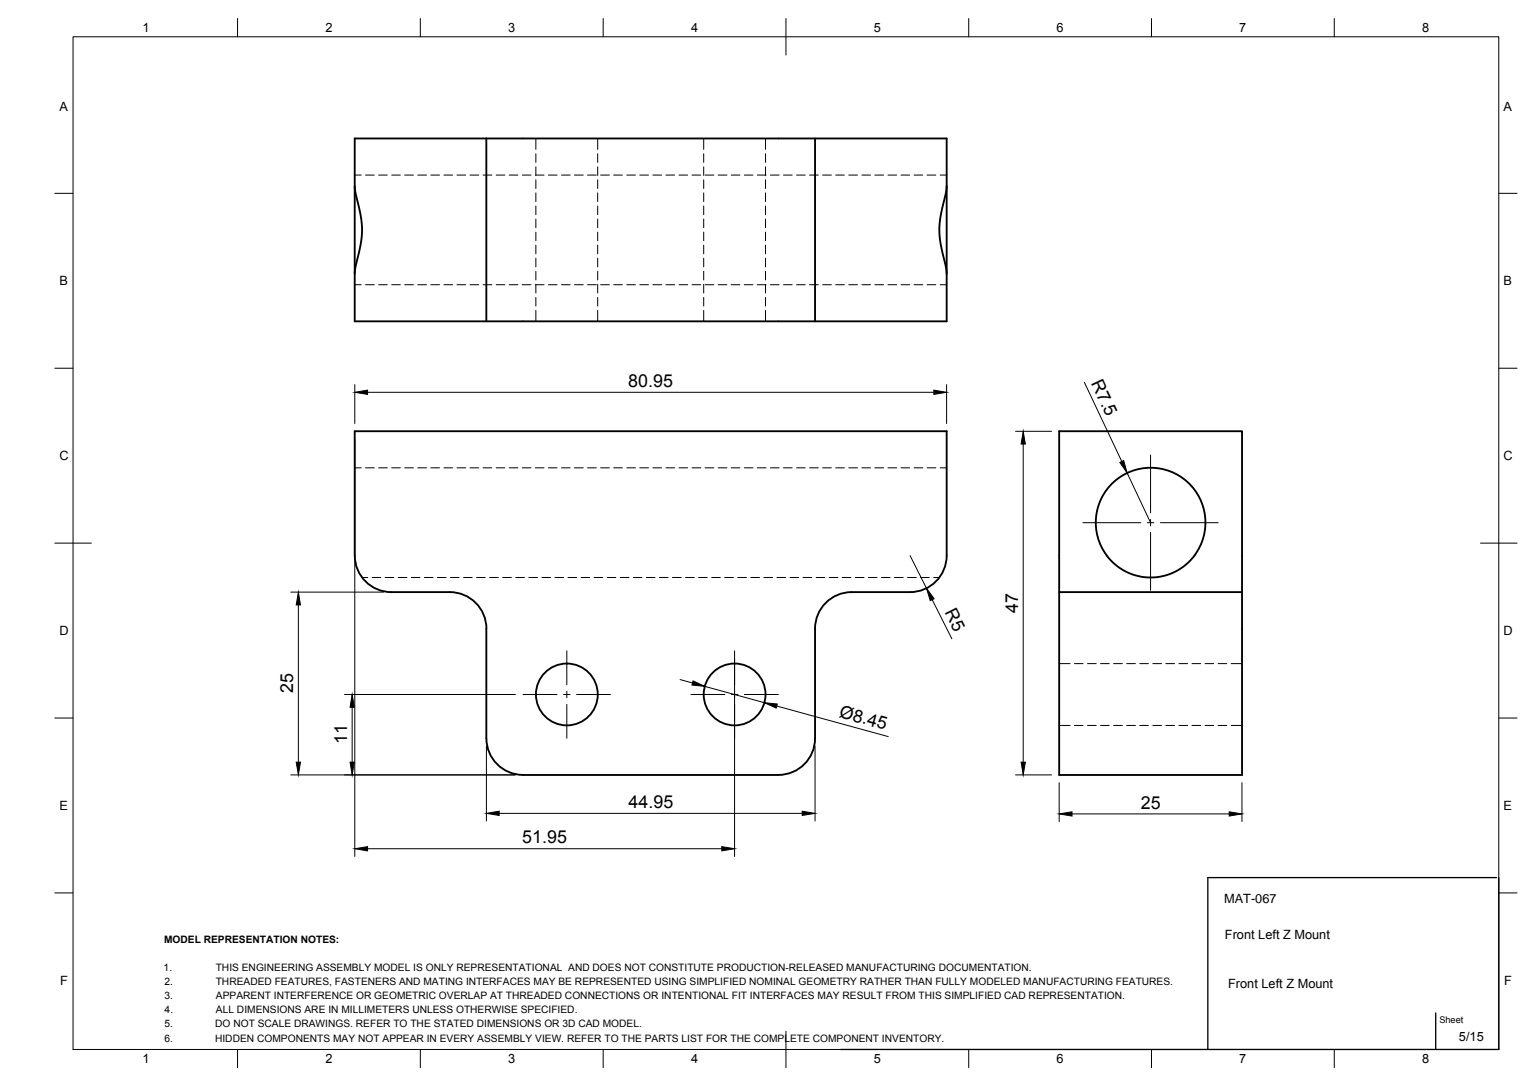
ISO-10303-21;
HEADER;
/* Generated by software containing ST-Developer
 * from STEP Tools, Inc. (www.steptools.com) 
 */

FILE_DESCRIPTION(
/* description */ ('CAx-IF Rec.Pracs.---Representation and Presentation of Product Manufa
cturing Information (PMI)---4.0---2014-10-13'),
/* implementation_level */ '2;1');

FILE_NAME(
/* name */ 'Front Left Z Mount.step',
/* time_stamp */ '2026-10-24T16:02:03-07:00',
/* author */ (''),
/* organization */ (''),
/* preprocessor_version */ 'ST-DEVELOPER v20.2',
/* originating_system */ 'Autodesk Translation Framework v15.17.0.0',
/* authorisation */ '');

FILE_SCHEMA (('AP242_MANAGED_MODEL_BASED_3D_ENGINEERING_MIM_LF { 1 0 10303 442 2 1 4 }'));
ENDSEC;

DATA;
#10=MECHANICAL_DESIGN_GEOMETRIC_PRESENTATION_REPRESENTATION('',(#351),#6348);
#329=SHAPE_REPRESENTATION_RELATIONSHIP('SRR','None',#6479,#340);
#340=ADVANCED_BREP_SHAPE_REPRESENTATION('',(#362),#6327);
#351=STYLED_ITEM('',(#6602),#362);
#362=MANIFOLD_SOLID_BREP('Body1',#3390);
#375=B_SPLINE_CURVE_WITH_KNOTS('',3,(#5524,#5525,#5526,#5527,#5528,#5529,
#5530,#5531,#5532,#5533,#5534,#5535,#5536,#5537,#5538,#5539,#5540,#5541),
 .UNSPECIFIED.,.F.,.F.,(4,2,2,2,2,2,2,2,4),(-2.14352388719531,-2.06484634554612,
-1.76300355616504,-1.61208216147449,-1.46116076678395,-1.31023937209341,
-1.15931797740286,-0.857475188021775,-0.778797646372586),.UNSPECIFIED.);
#376=B_SPLINE_CURVE_WITH_KNOTS('',3,(#5543,#5544,#5545,#5546,#5547,#5548,
#5549,#5550,#5551,#5552,#5553,#5554,#5555,#5556,#5557,#5558,#5559,#5560),
 .UNSPECIFIED.,.F.,.F.,(4,2,2,2,2,2,2,2,4),(-5.06584542076321,-4.98716787911402,
-4.68532508973293,-4.53440369504239,-4.38348230035184,-4.2325609056613,
-4.08163951097076,-3.77979672158967,-3.70111917994048),.UNSPECIFIED.);
#403=CYLINDRICAL_SURFACE('',#3628,0.004225);
#404=CYLINDRICAL_SURFACE('',#3629,0.004225);
#405=CYLINDRICAL_SURFACE('',#3631,0.0075);
#406=CYLINDRICAL_SURFACE('',#3636,0.005);
#407=CYLINDRICAL_SURFACE('',#3637,0.005);
#408=CYLINDRICAL_SURFACE('',#3638,0.005);
#409=CYLINDRICAL_SURFACE('',#3639,0.005);
#410=CYLINDRICAL_SURFACE('',#3640,0.005);
#411=CYLINDRICAL_SURFACE('',#3641,0.005);
#472=FACE_BOUND('',#915,.T.);
#473=FACE_BOUND('',#916,.T.);
#474=FACE_BOUND('',#918,.T.);
#475=FACE_BOUND('',#919,.T.);
#546=CIRCLE('',#3605,0.0075);
#547=CIRCLE('',#3606,0.0075);
#548=CIRCLE('',#3608,0.0075);
#549=CIRCLE('',#3609,0.0075);
#550=CIRCLE('',#3611,0.005);
#551=CIRCLE('',#3612,0.005);
#552=CIRCLE('',#3613,0.005);
#553=CIRCLE('',#3614,0.005);
#554=CIRCLE('',#3615,0.005);
#555=CIRCLE('',#3616,0.005);
#556=CIRCLE('',#3617,0.004225);
#557=CIRCLE('',#3618,0.004225);
#558=CIRCLE('',#3620,0.005);
#559=CIRCLE('',#3621,0.005);
#560=CIRCLE('',#3622,0.005);
#561=CIRCLE('',#3623,0.005);
#562=CIRCLE('',#3624,0.005);
#563=CIRCLE('',#3625,0.005);
#564=CIRCLE('',#3626,0.004225);
#565=CIRCLE('',#3627,0.004225);
#732=FACE_OUTER_BOUND('',#911,.T.);
#733=FACE_OUTER_BOUND('',#912,.T.);
#734=FACE_OUTER_BOUND('',#913,.T.);
#735=FACE_OUTER_BOUND('',#914,.T.);
#736=FACE_OUTER_BOUND('',#917,.T.);
#737=FACE_OUTER_BOUND('',#920,.T.);
#738=FACE_OUTER_BOUND('',#921,.T.);
#739=FACE_OUTER_BOUND('',#922,.T.);
#740=FACE_OUTER_BOUND('',#923,.T.);
#741=FACE_OUTER_BOUND('',#924,.T.);
#742=FACE_OUTER_BOUND('',#925,.T.);
#743=FACE_OUTER_BOUND('',#926,.T.);
#744=FACE_OUTER_BOUND('',#927,.T.);
#745=FACE_OUTER_BOUND('',#928,.T.);
#746=FACE_OUTER_BOUND('',#929,.T.);
#747=FACE_OUTER_BOUND('',#930,.T.);
#748=FACE_OUTER_BOUND('',#931,.T.);
#749=FACE_OUTER_BOUND('',#932,.T.);
#750=FACE_OUTER_BOUND('',#933,.T.);
#911=EDGE_LOOP('',(#2495,#2496,#2497,#2498));
#912=EDGE_LOOP('',(#2499,#2500,#2501,#2502,#2503,#2504,#2505));
#913=EDGE_LOOP('',(#2506,#2507,#2508,#2509,#2510,#2511,#2512));
#914=EDGE_LOOP('',(#2513,#2514,#2515,#2516,#2517,#2518,#2519,#2520,#2521,
#2522,#2523,#2524,#2525,#2526));
#915=EDGE_LOOP('',(#2527));
#916=EDGE_LOOP('',(#2528));
#917=EDGE_LOOP('',(#2529,#2530,#2531,#2532,#2533,#2534,#2535,#2536,#2537,
#2538,#2539,#2540,#2541,#2542));
#918=EDGE_LOOP('',(#2543));
#919=EDGE_LOOP('',(#2544));
#920=EDGE_LOOP('',(#2545,#2546,#2547,#2548));
#921=EDGE_LOOP('',(#2549,#2550,#2551,#2552));
#922=EDGE_LOOP('',(#2553,#2554,#2555,#2556));
#923=EDGE_LOOP('',(#2557,#2558,#2559,#2560,#2561,#2562,#2563,#2564));
#924=EDGE_LOOP('',(#2565,#2566,#2567,#2568));
#925=EDGE_LOOP('',(#2569,#2570,#2571,#2572));
#926=EDGE_LOOP('',(#2573,#2574,#2575,#2576));
#927=EDGE_LOOP('',(#2577,#2578,#2579,#2580));
#928=EDGE_LOOP('',(#2581,#2582,#2583,#2584));
#929=EDGE_LOOP('',(#2585,#2586,#2587,#2588,#2589,#2590));
#930=EDGE_LOOP('',(#2591,#2592,#2593,#2594));
#931=EDGE_LOOP('',(#2595,#2596,#2597,#2598,#2599,#2600));
#932=EDGE_LOOP('',(#2601,#2602,#2603,#2604));
#933=EDGE_LOOP('',(#2605,#2606,#2607,#2608));
#1148=LINE('',#5434,#1381);
#1149=LINE('',#5436,#1382);
#1150=LINE('',#5438,#1383);
#1151=LINE('',#5439,#1384);
#1152=LINE('',#5443,#1385);
#1153=LINE('',#5445,#1386);
#1154=LINE('',#5451,#1387);
#1155=LINE('',#5453,#1388);
#1156=LINE('',#5454,#1389);
#1157=LINE('',#5458,#1390);
#1158=LINE('',#5460,#1391);
#1159=LINE('',#5466,#1392);
#1160=LINE('',#5468,#1393);
#1161=LINE('',#5469,#1394);
#1162=LINE('',#5474,#1395);
#1163=LINE('',#5478,#1396);
#1164=LINE('',#5480,#1397);
#1165=LINE('',#5484,#1398);
#1166=LINE('',#5488,#1399);
#1167=LINE('',#5497,#1400);
#1168=LINE('',#5502,#1401);
#1169=LINE('',#5506,#1402);
#1170=LINE('',#5508,#1403);
#1171=LINE('',#5512,#1404);
#1172=LINE('',#5519,#1405);
#1173=LINE('',#5521,#1406);
#1174=LINE('',#5542,#1407);
#1175=LINE('',#5562,#1408);
#1176=LINE('',#5563,#1409);
#1177=LINE('',#5565,#1410);
#1178=LINE('',#5566,#1411);
#1179=LINE('',#5568,#1412);
#1180=LINE('',#5569,#1413);
#1181=LINE('',#5571,#1414);
#1182=LINE('',#5572,#1415);
#1381=VECTOR('',#4216,1.);
#1382=VECTOR('',#4217,1.);
#1383=VECTOR('',#4218,1.);
#1384=VECTOR('',#4219,1.);
#1385=VECTOR('',#4222,1.);
#1386=VECTOR('',#4223,1.);
#1387=VECTOR('',#4228,1.);
#1388=VECTOR('',#4229,1.);
#1389=VECTOR('',#4230,1.);
#1390=VECTOR('',#4233,1.);
#1391=VECTOR('',#4234,1.);
#1392=VECTOR('',#4239,1.);
#1393=VECTOR('',#4240,1.);
#1394=VECTOR('',#4241,1.);
#1395=VECTOR('',#4246,1.);
#1396=VECTOR('',#4249,1.);
#1397=VECTOR('',#4252,1.);
#1398=VECTOR('',#4255,1.);
#1399=VECTOR('',#4258,1.);
#1400=VECTOR('',#4267,1.);
#1401=VECTOR('',#4272,1.);
#1402=VECTOR('',#4275,1.);
#1403=VECTOR('',#4278,1.);
#1404=VECTOR('',#4281,1.);
#1405=VECTOR('',#4290,0.004225);
#1406=VECTOR('',#4293,0.004225);
#1407=VECTOR('',#4298,0.0075);
#1408=VECTOR('',#4301,1.);
#1409=VECTOR('',#4302,1.);
#1410=VECTOR('',#4305,1.);
#1411=VECTOR('',#4306,1.);
#1412=VECTOR('',#4309,1.);
#1413=VECTOR('',#4310,1.);
#1414=VECTOR('',#4313,1.);
#1415=VECTOR('',#4314,1.);
#1620=VERTEX_POINT('',#5432);
#1621=VERTEX_POINT('',#5433);
#1622=VERTEX_POINT('',#5435);
#1623=VERTEX_POINT('',#5437);
#1624=VERTEX_POINT('',#5441);
#1625=VERTEX_POINT('',#5442);
#1626=VERTEX_POINT('',#5444);
#1627=VERTEX_POINT('',#5446);
#1628=VERTEX_POINT('',#5448);
#1629=VERTEX_POINT('',#5450);
#1630=VERTEX_POINT('',#5452);
#1631=VERTEX_POINT('',#5456);
#1632=VERTEX_POINT('',#5457);
#1633=VERTEX_POINT('',#5459);
#1634=VERTEX_POINT('',#5461);
#1635=VERTEX_POINT('',#5463);
#1636=VERTEX_POINT('',#5465);
#1637=VERTEX_POINT('',#5467);
#1638=VERTEX_POINT('',#5471);
#1639=VERTEX_POINT('',#5473);
#1640=VERTEX_POINT('',#5475);
#1641=VERTEX_POINT('',#5477);
#1642=VERTEX_POINT('',#5481);
#1643=VERTEX_POINT('',#5483);
#1644=VERTEX_POINT('',#5485);
#1645=VERTEX_POINT('',#5487);
#1646=VERTEX_POINT('',#5490);
#1647=VERTEX_POINT('',#5492);
#1648=VERTEX_POINT('',#5495);
#1649=VERTEX_POINT('',#5496);
#1650=VERTEX_POINT('',#5499);
#1651=VERTEX_POINT('',#5501);
#1652=VERTEX_POINT('',#5503);
#1653=VERTEX_POINT('',#5505);
#1654=VERTEX_POINT('',#5509);
#1655=VERTEX_POINT('',#5511);
#1656=VERTEX_POINT('',#5514);
#1657=VERTEX_POINT('',#5516);
#1946=EDGE_CURVE('',#1620,#1621,#1148,.T.);
#1947=EDGE_CURVE('',#1621,#1622,#1149,.T.);
#1948=EDGE_CURVE('',#1623,#1622,#1150,.T.);
#1949=EDGE_CURVE('',#1623,#1620,#1151,.F.);
#1950=EDGE_CURVE('',#1624,#1625,#1152,.T.);
#1951=EDGE_CURVE('',#1624,#1626,#1153,.F.);
#1952=EDGE_CURVE('',#1626,#1627,#546,.T.);
#1953=EDGE_CURVE('',#1627,#1628,#547,.T.);
#1954=EDGE_CURVE('',#1628,#1629,#1154,.F.);
#1955=EDGE_CURVE('',#1629,#1630,#1155,.T.);
#1956=EDGE_CURVE('',#1625,#1630,#1156,.T.);
#1957=EDGE_CURVE('',#1631,#1632,#1157,.T.);
#1958=EDGE_CURVE('',#1631,#1633,#1158,.T.);
#1959=EDGE_CURVE('',#1634,#1633,#548,.T.);
#1960=EDGE_CURVE('',#1635,#1634,#549,.T.);
#1961=EDGE_CURVE('',#1635,#1636,#1159,.T.);
#1962=EDGE_CURVE('',#1636,#1637,#1160,.T.);
#1963=EDGE_CURVE('',#1637,#1632,#1161,.T.);
#1964=EDGE_CURVE('',#1622,#1638,#550,.T.);
#1965=EDGE_CURVE('',#1638,#1639,#1162,.T.);
#1966=EDGE_CURVE('',#1639,#1640,#551,.F.);
#1967=EDGE_CURVE('',#1641,#1640,#1163,.T.);
#1968=EDGE_CURVE('',#1641,#1624,#552,.T.);
#1969=EDGE_CURVE('',#1637,#1625,#1164,.T.);
#1970=EDGE_CURVE('',#1636,#1642,#553,.T.);
#1971=EDGE_CURVE('',#1642,#1643,#1165,.T.);
#1972=EDGE_CURVE('',#1643,#1644,#554,.F.);
#1973=EDGE_CURVE('',#1645,#1644,#1166,.T.);
#1974=EDGE_CURVE('',#1645,#1623,#555,.T.);
#1975=EDGE_CURVE('',#1646,#1646,#556,.T.);
#1976=EDGE_CURVE('',#1647,#1647,#557,.T.);
#1977=EDGE_CURVE('',#1648,#1649,#1167,.T.);
#1978=EDGE_CURVE('',#1648,#1621,#558,.F.);
#1979=EDGE_CURVE('',#1620,#1650,#559,.F.);
#1980=EDGE_CURVE('',#1650,#1651,#1168,.T.);
#1981=EDGE_CURVE('',#1651,#1652,#560,.T.);
#1982=EDGE_CURVE('',#1653,#1652,#1169,.T.);
#1983=EDGE_CURVE('',#1653,#1631,#561,.F.);
#1984=EDGE_CURVE('',#1632,#1630,#1170,.T.);
#1985=EDGE_CURVE('',#1629,#1654,#562,.F.);
#1986=EDGE_CURVE('',#1654,#1655,#1171,.T.);
#1987=EDGE_CURVE('',#1655,#1649,#563,.T.);
#1988=EDGE_CURVE('',#1656,#1656,#564,.T.);
#1989=EDGE_CURVE('',#1657,#1657,#565,.T.);
#1990=EDGE_CURVE('',#1646,#1656,#1172,.T.);
#1991=EDGE_CURVE('',#1647,#1657,#1173,.T.);
#1992=EDGE_CURVE('',#1626,#1628,#375,.T.);
#1993=EDGE_CURVE('',#1627,#1634,#1174,.T.);
#1994=EDGE_CURVE('',#1633,#1635,#376,.T.);
#1995=EDGE_CURVE('',#1638,#1648,#1175,.F.);
#1996=EDGE_CURVE('',#1649,#1639,#1176,.T.);
#1997=EDGE_CURVE('',#1654,#1641,#1177,.T.);
#1998=EDGE_CURVE('',#1640,#1655,#1178,.F.);
#1999=EDGE_CURVE('',#1644,#1651,#1179,.F.);
#2000=EDGE_CURVE('',#1650,#1645,#1180,.T.);
#2001=EDGE_CURVE('',#1642,#1653,#1181,.F.);
#2002=EDGE_CURVE('',#1652,#1643,#1182,.T.);
#2495=ORIENTED_EDGE('',*,*,#1946,.T.);
#2496=ORIENTED_EDGE('',*,*,#1947,.T.);
#2497=ORIENTED_EDGE('',*,*,#1948,.F.);
#2498=ORIENTED_EDGE('',*,*,#1949,.T.);
#2499=ORIENTED_EDGE('',*,*,#1950,.F.);
#2500=ORIENTED_EDGE('',*,*,#1951,.T.);
#2501=ORIENTED_EDGE('',*,*,#1952,.T.);
#2502=ORIENTED_EDGE('',*,*,#1953,.T.);
#2503=ORIENTED_EDGE('',*,*,#1954,.T.);
#2504=ORIENTED_EDGE('',*,*,#1955,.T.);
#2505=ORIENTED_EDGE('',*,*,#1956,.F.);
#2506=ORIENTED_EDGE('',*,*,#1957,.F.);
#2507=ORIENTED_EDGE('',*,*,#1958,.T.);
#2508=ORIENTED_EDGE('',*,*,#1959,.F.);
#2509=ORIENTED_EDGE('',*,*,#1960,.F.);
#2510=ORIENTED_EDGE('',*,*,#1961,.T.);
#2511=ORIENTED_EDGE('',*,*,#1962,.T.);
#2512=ORIENTED_EDGE('',*,*,#1963,.T.);
#2513=ORIENTED_EDGE('',*,*,#1948,.T.);
#2514=ORIENTED_EDGE('',*,*,#1964,.T.);
#2515=ORIENTED_EDGE('',*,*,#1965,.T.);
#2516=ORIENTED_EDGE('',*,*,#1966,.T.);
#2517=ORIENTED_EDGE('',*,*,#1967,.F.);
#2518=ORIENTED_EDGE('',*,*,#1968,.T.);
#2519=ORIENTED_EDGE('',*,*,#1950,.T.);
#2520=ORIENTED_EDGE('',*,*,#1969,.F.);
#2521=ORIENTED_EDGE('',*,*,#1962,.F.);
#2522=ORIENTED_EDGE('',*,*,#1970,.T.);
#2523=ORIENTED_EDGE('',*,*,#1971,.T.);
#2524=ORIENTED_EDGE('',*,*,#1972,.T.);
#2525=ORIENTED_EDGE('',*,*,#1973,.F.);
#2526=ORIENTED_EDGE('',*,*,#1974,.T.);
#2527=ORIENTED_EDGE('',*,*,#1975,.F.);
#2528=ORIENTED_EDGE('',*,*,#1976,.F.);
#2529=ORIENTED_EDGE('',*,*,#1977,.F.);
#2530=ORIENTED_EDGE('',*,*,#1978,.T.);
#2531=ORIENTED_EDGE('',*,*,#1946,.F.);
#2532=ORIENTED_EDGE('',*,*,#1979,.T.);
#2533=ORIENTED_EDGE('',*,*,#1980,.T.);
#2534=ORIENTED_EDGE('',*,*,#1981,.T.);
#2535=ORIENTED_EDGE('',*,*,#1982,.F.);
#2536=ORIENTED_EDGE('',*,*,#1983,.T.);
#2537=ORIENTED_EDGE('',*,*,#1957,.T.);
#2538=ORIENTED_EDGE('',*,*,#1984,.T.);
#2539=ORIENTED_EDGE('',*,*,#1955,.F.);
#2540=ORIENTED_EDGE('',*,*,#1985,.T.);
#2541=ORIENTED_EDGE('',*,*,#1986,.T.);
#2542=ORIENTED_EDGE('',*,*,#1987,.T.);
#2543=ORIENTED_EDGE('',*,*,#1988,.T.);
#2544=ORIENTED_EDGE('',*,*,#1989,.T.);
#2545=ORIENTED_EDGE('',*,*,#1975,.T.);
#2546=ORIENTED_EDGE('',*,*,#1990,.T.);
#2547=ORIENTED_EDGE('',*,*,#1988,.F.);
#2548=ORIENTED_EDGE('',*,*,#1990,.F.);
#2549=ORIENTED_EDGE('',*,*,#1976,.T.);
#2550=ORIENTED_EDGE('',*,*,#1991,.T.);
#2551=ORIENTED_EDGE('',*,*,#1989,.F.);
#2552=ORIENTED_EDGE('',*,*,#1991,.F.);
#2553=ORIENTED_EDGE('',*,*,#1984,.F.);
#2554=ORIENTED_EDGE('',*,*,#1963,.F.);
#2555=ORIENTED_EDGE('',*,*,#1969,.T.);
#2556=ORIENTED_EDGE('',*,*,#1956,.T.);
#2557=ORIENTED_EDGE('',*,*,#1952,.F.);
#2558=ORIENTED_EDGE('',*,*,#1992,.T.);
#2559=ORIENTED_EDGE('',*,*,#1953,.F.);
#2560=ORIENTED_EDGE('',*,*,#1993,.T.);
#2561=ORIENTED_EDGE('',*,*,#1959,.T.);
#2562=ORIENTED_EDGE('',*,*,#1994,.T.);
#2563=ORIENTED_EDGE('',*,*,#1960,.T.);
#2564=ORIENTED_EDGE('',*,*,#1993,.F.);
#2565=ORIENTED_EDGE('',*,*,#1965,.F.);
#2566=ORIENTED_EDGE('',*,*,#1995,.T.);
#2567=ORIENTED_EDGE('',*,*,#1977,.T.);
#2568=ORIENTED_EDGE('',*,*,#1996,.T.);
#2569=ORIENTED_EDGE('',*,*,#1986,.F.);
#2570=ORIENTED_EDGE('',*,*,#1997,.T.);
#2571=ORIENTED_EDGE('',*,*,#1967,.T.);
#2572=ORIENTED_EDGE('',*,*,#1998,.T.);
#2573=ORIENTED_EDGE('',*,*,#1973,.T.);
#2574=ORIENTED_EDGE('',*,*,#1999,.T.);
#2575=ORIENTED_EDGE('',*,*,#1980,.F.);
#2576=ORIENTED_EDGE('',*,*,#2000,.T.);
#2577=ORIENTED_EDGE('',*,*,#1971,.F.);
#2578=ORIENTED_EDGE('',*,*,#2001,.T.);
#2579=ORIENTED_EDGE('',*,*,#1982,.T.);
#2580=ORIENTED_EDGE('',*,*,#2002,.T.);
#2581=ORIENTED_EDGE('',*,*,#1978,.F.);
#2582=ORIENTED_EDGE('',*,*,#1995,.F.);
#2583=ORIENTED_EDGE('',*,*,#1964,.F.);
#2584=ORIENTED_EDGE('',*,*,#1947,.F.);
#2585=ORIENTED_EDGE('',*,*,#1992,.F.);
#2586=ORIENTED_EDGE('',*,*,#1951,.F.);
#2587=ORIENTED_EDGE('',*,*,#1968,.F.);
#2588=ORIENTED_EDGE('',*,*,#1997,.F.);
#2589=ORIENTED_EDGE('',*,*,#1985,.F.);
#2590=ORIENTED_EDGE('',*,*,#1954,.F.);
#2591=ORIENTED_EDGE('',*,*,#1987,.F.);
#2592=ORIENTED_EDGE('',*,*,#1998,.F.);
#2593=ORIENTED_EDGE('',*,*,#1966,.F.);
#2594=ORIENTED_EDGE('',*,*,#1996,.F.);
#2595=ORIENTED_EDGE('',*,*,#1983,.F.);
#2596=ORIENTED_EDGE('',*,*,#2001,.F.);
#2597=ORIENTED_EDGE('',*,*,#1970,.F.);
#2598=ORIENTED_EDGE('',*,*,#1961,.F.);
#2599=ORIENTED_EDGE('',*,*,#1994,.F.);
#2600=ORIENTED_EDGE('',*,*,#1958,.F.);
#2601=ORIENTED_EDGE('',*,*,#1981,.F.);
#2602=ORIENTED_EDGE('',*,*,#1999,.F.);
#2603=ORIENTED_EDGE('',*,*,#1972,.F.);
#2604=ORIENTED_EDGE('',*,*,#2002,.F.);
#2605=ORIENTED_EDGE('',*,*,#1979,.F.);
#2606=ORIENTED_EDGE('',*,*,#1949,.F.);
#2607=ORIENTED_EDGE('',*,*,#1974,.F.);
#2608=ORIENTED_EDGE('',*,*,#2000,.F.);
#3157=PLANE('',#3603);
#3158=PLANE('',#3604);
#3159=PLANE('',#3607);
#3160=PLANE('',#3610);
#3161=PLANE('',#3619);
#3162=PLANE('',#3630);
#3163=PLANE('',#3632);
#3164=PLANE('',#3633);
#3165=PLANE('',#3634);
#3166=PLANE('',#3635);
#3255=ADVANCED_FACE('',(#732),#3157,.F.);
#3256=ADVANCED_FACE('',(#733),#3158,.F.);
#3257=ADVANCED_FACE('',(#734),#3159,.T.);
#3258=ADVANCED_FACE('',(#735,#472,#473),#3160,.T.);
#3259=ADVANCED_FACE('',(#736,#474,#475),#3161,.F.);
#3260=ADVANCED_FACE('',(#737),#403,.F.);
#3261=ADVANCED_FACE('',(#738),#404,.F.);
#3262=ADVANCED_FACE('',(#739),#3162,.T.);
#3263=ADVANCED_FACE('',(#740),#405,.F.);
#3264=ADVANCED_FACE('',(#741),#3163,.T.);
#3265=ADVANCED_FACE('',(#742),#3164,.F.);
#3266=ADVANCED_FACE('',(#743),#3165,.F.);
#3267=ADVANCED_FACE('',(#744),#3166,.T.);
#3268=ADVANCED_FACE('',(#745),#406,.T.);
#3269=ADVANCED_FACE('',(#746),#407,.T.);
#3270=ADVANCED_FACE('',(#747),#408,.F.);
#3271=ADVANCED_FACE('',(#748),#409,.T.);
#3272=ADVANCED_FACE('',(#749),#410,.F.);
#3273=ADVANCED_FACE('',(#750),#411,.T.);
#3390=CLOSED_SHELL('',(#3255,#3256,#3257,#3258,#3259,#3260,#3261,#3262,
#3263,#3264,#3265,#3266,#3267,#3268,#3269,#3270,#3271,#3272,#3273));
#3602=AXIS2_PLACEMENT_3D('',#5430,#4212,#4213);
#3603=AXIS2_PLACEMENT_3D('',#5431,#4214,#4215);
#3604=AXIS2_PLACEMENT_3D('',#5440,#4220,#4221);
#3605=AXIS2_PLACEMENT_3D('',#5447,#4224,#4225);
#3606=AXIS2_PLACEMENT_3D('',#5449,#4226,#4227);
#3607=AXIS2_PLACEMENT_3D('',#5455,#4231,#4232);
#3608=AXIS2_PLACEMENT_3D('',#5462,#4235,#4236);
#3609=AXIS2_PLACEMENT_3D('',#5464,#4237,#4238);
#3610=AXIS2_PLACEMENT_3D('',#5470,#4242,#4243);
#3611=AXIS2_PLACEMENT_3D('',#5472,#4244,#4245);
#3612=AXIS2_PLACEMENT_3D('',#5476,#4247,#4248);
#3613=AXIS2_PLACEMENT_3D('',#5479,#4250,#4251);
#3614=AXIS2_PLACEMENT_3D('',#5482,#4253,#4254);
#3615=AXIS2_PLACEMENT_3D('',#5486,#4256,#4257);
#3616=AXIS2_PLACEMENT_3D('',#5489,#4259,#4260);
#3617=AXIS2_PLACEMENT_3D('',#5491,#4261,#4262);
#3618=AXIS2_PLACEMENT_3D('',#5493,#4263,#4264);
#3619=AXIS2_PLACEMENT_3D('',#5494,#4265,#4266);
#3620=AXIS2_PLACEMENT_3D('',#5498,#4268,#4269);
#3621=AXIS2_PLACEMENT_3D('',#5500,#4270,#4271);
#3622=AXIS2_PLACEMENT_3D('',#5504,#4273,#4274);
#3623=AXIS2_PLACEMENT_3D('',#5507,#4276,#4277);
#3624=AXIS2_PLACEMENT_3D('',#5510,#4279,#4280);
#3625=AXIS2_PLACEMENT_3D('',#5513,#4282,#4283);
#3626=AXIS2_PLACEMENT_3D('',#5515,#4284,#4285);
#3627=AXIS2_PLACEMENT_3D('',#5517,#4286,#4287);
#3628=AXIS2_PLACEMENT_3D('',#5518,#4288,#4289);
#3629=AXIS2_PLACEMENT_3D('',#5520,#4291,#4292);
#3630=AXIS2_PLACEMENT_3D('',#5522,#4294,#4295);
#3631=AXIS2_PLACEMENT_3D('',#5523,#4296,#4297);
#3632=AXIS2_PLACEMENT_3D('',#5561,#4299,#4300);
#3633=AXIS2_PLACEMENT_3D('',#5564,#4303,#4304);
#3634=AXIS2_PLACEMENT_3D('',#5567,#4307,#4308);
#3635=AXIS2_PLACEMENT_3D('',#5570,#4311,#4312);
#3636=AXIS2_PLACEMENT_3D('',#5573,#4315,#4316);
#3637=AXIS2_PLACEMENT_3D('',#5574,#4317,#4318);
#3638=AXIS2_PLACEMENT_3D('',#5575,#4319,#4320);
#3639=AXIS2_PLACEMENT_3D('',#5576,#4321,#4322);
#3640=AXIS2_PLACEMENT_3D('',#5577,#4323,#4324);
#3641=AXIS2_PLACEMENT_3D('',#5578,#4325,#4326);
#4212=DIRECTION('axis',(0.,0.,1.));
#4213=DIRECTION('refdir',(1.,0.,0.));
#4214=DIRECTION('center_axis',(1.,0.,0.));
#4215=DIRECTION('ref_axis',(0.,0.,-1.));
#4216=DIRECTION('',(0.,-8.57182693503055E-17,-1.));
#4217=DIRECTION('',(0.,-1.,8.57182693503055E-17));
#4218=DIRECTION('',(0.,-8.57182693503055E-17,-1.));
#4219=DIRECTION('',(0.,-1.,8.57182693503055E-17));
#4220=DIRECTION('center_axis',(0.,8.57182693503055E-17,1.));
#4221=DIRECTION('ref_axis',(0.,-1.,8.57182693503055E-17));
#4222=DIRECTION('',(1.,0.,0.));
#4223=DIRECTION('',(0.,-1.,8.57182693503055E-17));
#4224=DIRECTION('center_axis',(0.,8.57182693503055E-17,1.));
#4225=DIRECTION('ref_axis',(0.,-1.,8.57182693503055E-17));
#4226=DIRECTION('center_axis',(0.,8.57182693503055E-17,1.));
#4227=DIRECTION('ref_axis',(0.,-1.,8.57182693503055E-17));
#4228=DIRECTION('',(0.,-1.,8.57182693503055E-17));
#4229=DIRECTION('',(1.,0.,0.));
#4230=DIRECTION('',(0.,1.,-8.57182693503055E-17));
#4231=DIRECTION('center_axis',(0.,8.57182693503055E-17,1.));
#4232=DIRECTION('ref_axis',(0.,-1.,8.57182693503055E-17));
#4233=DIRECTION('',(1.,0.,0.));
#4234=DIRECTION('',(0.,-1.,8.57182693503055E-17));
#4235=DIRECTION('center_axis',(0.,8.57182693503055E-17,1.));
#4236=DIRECTION('ref_axis',(0.,-1.,8.57182693503055E-17));
#4237=DIRECTION('center_axis',(0.,8.57182693503055E-17,1.));
#4238=DIRECTION('ref_axis',(0.,-1.,8.57182693503055E-17));
#4239=DIRECTION('',(0.,-1.,8.57182693503055E-17));
#4240=DIRECTION('',(1.,0.,0.));
#4241=DIRECTION('',(0.,1.,-8.57182693503055E-17));
#4242=DIRECTION('center_axis',(0.,-1.,8.57182693503055E-17));
#4243=DIRECTION('ref_axis',(1.,0.,0.));
#4244=DIRECTION('center_axis',(0.,-1.,8.57182693503055E-17));
#4245=DIRECTION('ref_axis',(0.,-8.57182693503055E-17,-1.));
#4246=DIRECTION('',(1.,0.,0.));
#4247=DIRECTION('center_axis',(0.,-1.,8.57182693503055E-17));
#4248=DIRECTION('ref_axis',(0.,-8.57182693503055E-17,-1.));
#4249=DIRECTION('',(0.,8.57182693503055E-17,1.));
#4250=DIRECTION('center_axis',(0.,-1.,8.57182693503055E-17));
#4251=DIRECTION('ref_axis',(0.,-8.57182693503055E-17,-1.));
#4252=DIRECTION('',(0.,-8.57182693503055E-17,-1.));
#4253=DIRECTION('center_axis',(0.,-1.,8.57182693503055E-17));
#4254=DIRECTION('ref_axis',(0.,-8.57182693503055E-17,-1.));
#4255=DIRECTION('',(0.,-8.57182693503055E-17,-1.));
#4256=DIRECTION('center_axis',(0.,-1.,8.57182693503055E-17));
#4257=DIRECTION('ref_axis',(0.,-8.57182693503055E-17,-1.));
#4258=DIRECTION('',(1.,0.,0.));
#4259=DIRECTION('center_axis',(0.,-1.,8.57182693503055E-17));
#4260=DIRECTION('ref_axis',(0.,-8.57182693503055E-17,-1.));
#4261=DIRECTION('center_axis',(0.,-1.,8.57182693503055E-17));
#4262=DIRECTION('ref_axis',(0.,-8.57182693503055E-17,-1.));
#4263=DIRECTION('center_axis',(0.,-1.,8.57182693503055E-17));
#4264=DIRECTION('ref_axis',(0.,-8.57182693503055E-17,-1.));
#4265=DIRECTION('center_axis',(0.,-1.,8.57182693503055E-17));
#4266=DIRECTION('ref_axis',(1.,0.,0.));
#4267=DIRECTION('',(1.,0.,0.));
#4268=DIRECTION('center_axis',(0.,-1.,8.57182693503055E-17));
#4269=DIRECTION('ref_axis',(0.,-8.57182693503055E-17,-1.));
#4270=DIRECTION('center_axis',(0.,-1.,8.57182693503055E-17));
#4271=DIRECTION('ref_axis',(0.,-8.57182693503055E-17,-1.));
#4272=DIRECTION('',(1.,0.,0.));
#4273=DIRECTION('center_axis',(0.,-1.,8.57182693503055E-17));
#4274=DIRECTION('ref_axis',(0.,-8.57182693503055E-17,-1.));
#4275=DIRECTION('',(0.,-8.57182693503055E-17,-1.));
#4276=DIRECTION('center_axis',(0.,-1.,8.57182693503055E-17));
#4277=DIRECTION('ref_axis',(0.,-8.57182693503055E-17,-1.));
#4278=DIRECTION('',(0.,-8.57182693503055E-17,-1.));
#4279=DIRECTION('center_axis',(0.,-1.,8.57182693503055E-17));
#4280=DIRECTION('ref_axis',(0.,-8.57182693503055E-17,-1.));
#4281=DIRECTION('',(0.,8.57182693503055E-17,1.));
#4282=DIRECTION('center_axis',(0.,-1.,8.57182693503055E-17));
#4283=DIRECTION('ref_axis',(0.,-8.57182693503055E-17,-1.));
#4284=DIRECTION('center_axis',(0.,-1.,8.57182693503055E-17));
#4285=DIRECTION('ref_axis',(0.,-8.57182693503055E-17,-1.));
#4286=DIRECTION('center_axis',(0.,-1.,8.57182693503055E-17));
#4287=DIRECTION('ref_axis',(0.,-8.57182693503055E-17,-1.));
#4288=DIRECTION('center_axis',(0.,1.,-8.57182693503055E-17));
#4289=DIRECTION('ref_axis',(0.,8.57182693503055E-17,1.));
#4290=DIRECTION('',(0.,1.,-8.57182693503055E-17));
#4291=DIRECTION('center_axis',(0.,1.,-8.57182693503055E-17));
#4292=DIRECTION('ref_axis',(0.,8.57182693503055E-17,1.));
#4293=DIRECTION('',(0.,1.,-8.57182693503055E-17));
#4294=DIRECTION('center_axis',(1.,0.,0.));
#4295=DIRECTION('ref_axis',(0.,0.,-1.));
#4296=DIRECTION('center_axis',(0.,8.57182693503055E-17,1.));
#4297=DIRECTION('ref_axis',(0.,-1.,8.57182693503055E-17));
#4298=DIRECTION('',(0.,8.57182693503055E-17,1.));
#4299=DIRECTION('center_axis',(0.,-8.57182693503055E-17,-1.));
#4300=DIRECTION('ref_axis',(0.,1.,-8.57182693503055E-17));
#4301=DIRECTION('',(0.,-1.,8.57182693503055E-17));
#4302=DIRECTION('',(0.,-1.,8.57182693503055E-17));
#4303=DIRECTION('center_axis',(1.,0.,0.));
#4304=DIRECTION('ref_axis',(0.,0.,-1.));
#4305=DIRECTION('',(0.,-1.,8.57182693503055E-17));
#4306=DIRECTION('',(0.,-1.,8.57182693503055E-17));
#4307=DIRECTION('center_axis',(0.,-8.57182693503055E-17,-1.));
#4308=DIRECTION('ref_axis',(0.,1.,-8.57182693503055E-17));
#4309=DIRECTION('',(0.,-1.,8.57182693503055E-17));
#4310=DIRECTION('',(0.,-1.,8.57182693503055E-17));
#4311=DIRECTION('center_axis',(-1.,0.,0.));
#4312=DIRECTION('ref_axis',(0.,0.,1.));
#4313=DIRECTION('',(0.,-1.,8.57182693503055E-17));
#4314=DIRECTION('',(0.,-1.,8.57182693503055E-17));
#4315=DIRECTION('center_axis',(0.,1.,-8.57182693503055E-17));
#4316=DIRECTION('ref_axis',(0.,8.57182693503055E-17,1.));
#4317=DIRECTION('center_axis',(0.,-1.,8.57182693503055E-17));
#4318=DIRECTION('ref_axis',(0.,-8.57182693503055E-17,-1.));
#4319=DIRECTION('center_axis',(0.,-1.,8.57182693503055E-17));
#4320=DIRECTION('ref_axis',(0.,-8.57182693503055E-17,-1.));
#4321=DIRECTION('center_axis',(0.,-1.,8.57182693503055E-17));
#4322=DIRECTION('ref_axis',(0.,-8.57182693503055E-17,-1.));
#4323=DIRECTION('center_axis',(0.,-1.,8.57182693503055E-17));
#4324=DIRECTION('ref_axis',(0.,-8.57182693503055E-17,-1.));
#4325=DIRECTION('center_axis',(0.,-1.,8.57182693503055E-17));
#4326=DIRECTION('ref_axis',(0.,-8.57182693503055E-17,-1.));
#5430=CARTESIAN_POINT('',(0.,0.,0.));
#5431=CARTESIAN_POINT('Origin',(-0.06855,-0.1092,0.02565));
#5432=CARTESIAN_POINT('',(-0.06855,-0.0842,0.043125));
#5433=CARTESIAN_POINT('',(-0.06855,-0.0842,0.008175));
#5434=CARTESIAN_POINT('',(-0.06855,-0.0842,0.02565));
#5435=CARTESIAN_POINT('',(-0.06855,-0.1092,0.008175));
#5436=CARTESIAN_POINT('',(-0.06855,-0.1092,0.008175));
#5437=CARTESIAN_POINT('',(-0.06855,-0.1092,0.043125));
#5438=CARTESIAN_POINT('',(-0.06855,-0.1092,0.02565));
#5439=CARTESIAN_POINT('',(-0.06855,-0.1092,0.043125));
#5440=CARTESIAN_POINT('Origin',(-0.05755,-0.1092,-0.014825));
#5441=CARTESIAN_POINT('',(-0.03855,-0.1092,-0.014825));
#5442=CARTESIAN_POINT('',(-0.02155,-0.1092,-0.014825));
#5443=CARTESIAN_POINT('',(-0.05755,-0.1092,-0.014825));
#5444=CARTESIAN_POINT('',(-0.03855,-0.1027,-0.014825));
#5445=CARTESIAN_POINT('',(-0.03855,-0.1092,-0.014825));
#5446=CARTESIAN_POINT('',(-0.03405,-0.0892,-0.014825));
#5447=CARTESIAN_POINT('Origin',(-0.03405,-0.0967,-0.014825));
#5448=CARTESIAN_POINT('',(-0.03855,-0.0907,-0.014825));
#5449=CARTESIAN_POINT('Origin',(-0.03405,-0.0967,-0.014825));
#5450=CARTESIAN_POINT('',(-0.03855,-0.0842,-0.014825));
#5451=CARTESIAN_POINT('',(-0.03855,-0.1092,-0.014825));
#5452=CARTESIAN_POINT('',(-0.02155,-0.0842,-0.014825));
#5453=CARTESIAN_POINT('',(-0.05755,-0.0842,-0.014825));
#5454=CARTESIAN_POINT('',(-0.02155,-0.1092,-0.014825));
#5455=CARTESIAN_POINT('Origin',(-0.05755,-0.1092,0.066125));
#5456=CARTESIAN_POINT('',(-0.03855,-0.0842,0.066125));
#5457=CARTESIAN_POINT('',(-0.02155,-0.0842,0.066125));
#5458=CARTESIAN_POINT('',(-0.05755,-0.0842,0.066125));
#5459=CARTESIAN_POINT('',(-0.03855,-0.0907,0.066125));
#5460=CARTESIAN_POINT('',(-0.03855,-0.1092,0.066125));
#5461=CARTESIAN_POINT('',(-0.03405,-0.0892,0.066125));
#5462=CARTESIAN_POINT('Origin',(-0.03405,-0.0967,0.066125));
#5463=CARTESIAN_POINT('',(-0.03855,-0.1027,0.066125));
#5464=CARTESIAN_POINT('Origin',(-0.03405,-0.0967,0.066125));
#5465=CARTESIAN_POINT('',(-0.03855,-0.1092,0.066125));
#5466=CARTESIAN_POINT('',(-0.03855,-0.1092,0.066125));
#5467=CARTESIAN_POINT('',(-0.02155,-0.1092,0.066125));
#5468=CARTESIAN_POINT('',(-0.05755,-0.1092,0.066125));
#5469=CARTESIAN_POINT('',(-0.02155,-0.1092,0.066125));
#5470=CARTESIAN_POINT('Origin',(-0.05755,-0.1092,0.02565));
#5471=CARTESIAN_POINT('',(-0.06355,-0.1092,0.003175));
#5472=CARTESIAN_POINT('Origin',(-0.06355,-0.1092,0.008175));
#5473=CARTESIAN_POINT('',(-0.04855,-0.1092,0.003175));
#5474=CARTESIAN_POINT('',(-0.05605,-0.1092,0.003175));
#5475=CARTESIAN_POINT('',(-0.04355,-0.1092,-0.001825));
#5476=CARTESIAN_POINT('Origin',(-0.04855,-0.1092,-0.001825));
#5477=CARTESIAN_POINT('',(-0.04355,-0.1092,-0.009825));
#5478=CARTESIAN_POINT('',(-0.04355,-0.1092,-0.005825));
#5479=CARTESIAN_POINT('Origin',(-0.03855,-0.1092,-0.009825));
#5480=CARTESIAN_POINT('',(-0.02155,-0.1092,0.02565));
#5481=CARTESIAN_POINT('',(-0.04355,-0.1092,0.061125));
#5482=CARTESIAN_POINT('Origin',(-0.03855,-0.1092,0.061125));
#5483=CARTESIAN_POINT('',(-0.04355,-0.1092,0.053125));
#5484=CARTESIAN_POINT('',(-0.04355,-0.1092,0.057125));
#5485=CARTESIAN_POINT('',(-0.04855,-0.1092,0.048125));
#5486=CARTESIAN_POINT('Origin',(-0.04855,-0.1092,0.053125));
#5487=CARTESIAN_POINT('',(-0.06355,-0.1092,0.048125));
#5488=CARTESIAN_POINT('',(-0.05605,-0.1092,0.048125));
#5489=CARTESIAN_POINT('Origin',(-0.06355,-0.1092,0.043125));
#5490=CARTESIAN_POINT('',(-0.05755,-0.1092,0.0329));
#5491=CARTESIAN_POINT('Origin',(-0.05755,-0.1092,0.037125));
#5492=CARTESIAN_POINT('',(-0.05755,-0.1092,0.00995));
#5493=CARTESIAN_POINT('Origin',(-0.05755,-0.1092,0.014175));
#5494=CARTESIAN_POINT('Origin',(-0.05755,-0.0842,0.02565));
#5495=CARTESIAN_POINT('',(-0.06355,-0.0842,0.003175));
#5496=CARTESIAN_POINT('',(-0.04855,-0.0842,0.003175));
#5497=CARTESIAN_POINT('',(-0.05605,-0.0842,0.003175));
#5498=CARTESIAN_POINT('Origin',(-0.06355,-0.0842,0.008175));
#5499=CARTESIAN_POINT('',(-0.06355,-0.0842,0.048125));
#5500=CARTESIAN_POINT('Origin',(-0.06355,-0.0842,0.043125));
#5501=CARTESIAN_POINT('',(-0.04855,-0.0842,0.048125));
#5502=CARTESIAN_POINT('',(-0.05605,-0.0842,0.048125));
#5503=CARTESIAN_POINT('',(-0.04355,-0.0842,0.053125));
#5504=CARTESIAN_POINT('Origin',(-0.04855,-0.0842,0.053125));
#5505=CARTESIAN_POINT('',(-0.04355,-0.0842,0.061125));
#5506=CARTESIAN_POINT('',(-0.04355,-0.0842,0.057125));
#5507=CARTESIAN_POINT('Origin',(-0.03855,-0.0842,0.061125));
#5508=CARTESIAN_POINT('',(-0.02155,-0.0842,0.02565));
#5509=CARTESIAN_POINT('',(-0.04355,-0.0842,-0.009825));
#5510=CARTESIAN_POINT('Origin',(-0.03855,-0.0842,-0.009825));
#5511=CARTESIAN_POINT('',(-0.04355,-0.0842,-0.001825));
#5512=CARTESIAN_POINT('',(-0.04355,-0.0842,-0.005825));
#5513=CARTESIAN_POINT('Origin',(-0.04855,-0.0842,-0.001825));
#5514=CARTESIAN_POINT('',(-0.05755,-0.0842,0.0329));
#5515=CARTESIAN_POINT('Origin',(-0.05755,-0.0842,0.037125));
#5516=CARTESIAN_POINT('',(-0.05755,-0.0842,0.00995));
#5517=CARTESIAN_POINT('Origin',(-0.05755,-0.0842,0.014175));
#5518=CARTESIAN_POINT('Origin',(-0.05755,-0.1092,0.037125));
#5519=CARTESIAN_POINT('',(-0.05755,-0.1092,0.0329));
#5520=CARTESIAN_POINT('Origin',(-0.05755,-0.1092,0.014175));
#5521=CARTESIAN_POINT('',(-0.05755,-0.1092,0.00995));
#5522=CARTESIAN_POINT('Origin',(-0.02155,-0.1092,0.02565));
#5523=CARTESIAN_POINT('Origin',(-0.03405,-0.0967,-0.023875));
#5524=CARTESIAN_POINT('Ctrl Pts',(-0.03855,-0.1027,-0.014825));
#5525=CARTESIAN_POINT('Ctrl Pts',(-0.0387729524989471,-0.10253278562579,
-0.014825));
#5526=CARTESIAN_POINT('Ctrl Pts',(-0.0389827504953742,-0.102355632371189,
-0.0148099450879691));
#5527=CARTESIAN_POINT('Ctrl Pts',(-0.0399051826894431,-0.101492776063005,
-0.0146940175331532));
#5528=CARTESIAN_POINT('Ctrl Pts',(-0.0405168708018142,-0.100636070492068,
-0.0144455865368071));
#5529=CARTESIAN_POINT('Ctrl Pts',(-0.0411335425015076,-0.0992177720348636,
-0.0141121811456859));
#5530=CARTESIAN_POINT('Ctrl Pts',(-0.0412904479475092,-0.0987224751365548,
-0.0140090151899698));
#5531=CARTESIAN_POINT('Ctrl Pts',(-0.0414987473161672,-0.0977152118956436,
-0.013864916792468));
#5532=CARTESIAN_POINT('Ctrl Pts',(-0.04155,-0.0972030713156352,-0.013825));
#5533=CARTESIAN_POINT('Ctrl Pts',(-0.04155,-0.0961969286843648,-0.013825));
#5534=CARTESIAN_POINT('Ctrl Pts',(-0.0414987473161672,-0.0956847881043564,
-0.013864916792468));
#5535=CARTESIAN_POINT('Ctrl Pts',(-0.0412904479475093,-0.0946775248634452,
-0.0140090151899698));
#5536=CARTESIAN_POINT('Ctrl Pts',(-0.0411335425015076,-0.0941822279651364,
-0.0141121811456859));
#5537=CARTESIAN_POINT('Ctrl Pts',(-0.0405168708018142,-0.0927639295079321,
-0.0144455865368071));
#5538=CARTESIAN_POINT('Ctrl Pts',(-0.0399051826894431,-0.0919072239369945,
-0.0146940175331532));
#5539=CARTESIAN_POINT('Ctrl Pts',(-0.0389827504953742,-0.0910443676288105,
-0.0148099450879691));
#5540=CARTESIAN_POINT('Ctrl Pts',(-0.0387729524989471,-0.0908672143742103,
-0.014825));
#5541=CARTESIAN_POINT('Ctrl Pts',(-0.03855,-0.0907,-0.014825));
#5542=CARTESIAN_POINT('',(-0.03405,-0.0892,-0.023875));
#5543=CARTESIAN_POINT('Ctrl Pts',(-0.03855,-0.0907,0.066125));
#5544=CARTESIAN_POINT('Ctrl Pts',(-0.0387729524989471,-0.0908672143742103,
0.066125));
#5545=CARTESIAN_POINT('Ctrl Pts',(-0.0389827504953742,-0.0910443676288105,
0.0661099450879691));
#5546=CARTESIAN_POINT('Ctrl Pts',(-0.039905182689443,-0.0919072239369945,
0.0659940175331532));
#5547=CARTESIAN_POINT('Ctrl Pts',(-0.0405168708018142,-0.0927639295079321,
0.0657455865368071));
#5548=CARTESIAN_POINT('Ctrl Pts',(-0.0411335425015076,-0.0941822279651364,
0.0654121811456859));
#5549=CARTESIAN_POINT('Ctrl Pts',(-0.0412904479475093,-0.0946775248634452,
0.0653090151899698));
#5550=CARTESIAN_POINT('Ctrl Pts',(-0.0414987473161672,-0.0956847881043564,
0.065164916792468));
#5551=CARTESIAN_POINT('Ctrl Pts',(-0.04155,-0.0961969286843649,0.065125));
#5552=CARTESIAN_POINT('Ctrl Pts',(-0.04155,-0.0972030713156351,0.065125));
#5553=CARTESIAN_POINT('Ctrl Pts',(-0.0414987473161672,-0.0977152118956436,
0.065164916792468));
#5554=CARTESIAN_POINT('Ctrl Pts',(-0.0412904479475092,-0.0987224751365548,
0.0653090151899699));
#5555=CARTESIAN_POINT('Ctrl Pts',(-0.0411335425015076,-0.0992177720348636,
0.0654121811456859));
#5556=CARTESIAN_POINT('Ctrl Pts',(-0.0405168708018142,-0.100636070492068,
0.0657455865368071));
#5557=CARTESIAN_POINT('Ctrl Pts',(-0.0399051826894431,-0.101492776063005,
0.0659940175331532));
#5558=CARTESIAN_POINT('Ctrl Pts',(-0.0389827504953742,-0.102355632371189,
0.0661099450879691));
#5559=CARTESIAN_POINT('Ctrl Pts',(-0.0387729524989471,-0.10253278562579,
0.066125));
#5560=CARTESIAN_POINT('Ctrl Pts',(-0.03855,-0.1027,0.066125));
#5561=CARTESIAN_POINT('Origin',(-0.05605,-0.0842,0.003175));
#5562=CARTESIAN_POINT('',(-0.06355,-0.0842,0.003175));
#5563=CARTESIAN_POINT('',(-0.04855,-0.0842,0.003175));
#5564=CARTESIAN_POINT('Origin',(-0.04355,-0.0842,-0.005825));
#5565=CARTESIAN_POINT('',(-0.04355,-0.0842,-0.009825));
#5566=CARTESIAN_POINT('',(-0.04355,-0.0842,-0.001825));
#5567=CARTESIAN_POINT('Origin',(-0.05605,-0.0842,0.048125));
#5568=CARTESIAN_POINT('',(-0.04855,-0.0842,0.048125));
#5569=CARTESIAN_POINT('',(-0.06355,-0.0842,0.048125));
#5570=CARTESIAN_POINT('Origin',(-0.04355,-0.0842,0.057125));
#5571=CARTESIAN_POINT('',(-0.04355,-0.0842,0.061125));
#5572=CARTESIAN_POINT('',(-0.04355,-0.0842,0.053125));
#5573=CARTESIAN_POINT('Origin',(-0.06355,-0.1092,0.008175));
#5574=CARTESIAN_POINT('Origin',(-0.03855,-0.0842,-0.009825));
#5575=CARTESIAN_POINT('Origin',(-0.04855,-0.0842,-0.001825));
#5576=CARTESIAN_POINT('Origin',(-0.03855,-0.1092,0.061125));
#5577=CARTESIAN_POINT('Origin',(-0.04855,-0.0842,0.053125));
#5578=CARTESIAN_POINT('Origin',(-0.06355,-0.0842,0.043125));
#6302=UNCERTAINTY_MEASURE_WITH_UNIT(LENGTH_MEASURE(1.E-5),#6349,
'DISTANCE_ACCURACY_VALUE',
'Maximum model space distance between geometric entities at asserted c
onnectivities');
#6323=UNCERTAINTY_MEASURE_WITH_UNIT(LENGTH_MEASURE(1.E-5),#6349,
'DISTANCE_ACCURACY_VALUE',
'Maximum model space distance between geometric entities at asserted c
onnectivities');
#6327=(
GEOMETRIC_REPRESENTATION_CONTEXT(3)
GLOBAL_UNCERTAINTY_ASSIGNED_CONTEXT((#6302))
GLOBAL_UNIT_ASSIGNED_CONTEXT((#6349,#6350,#6351))
REPRESENTATION_CONTEXT('','3D')
);
#6348=(
GEOMETRIC_REPRESENTATION_CONTEXT(3)
GLOBAL_UNCERTAINTY_ASSIGNED_CONTEXT((#6323))
GLOBAL_UNIT_ASSIGNED_CONTEXT((#6349,#6350,#6351))
REPRESENTATION_CONTEXT('','3D')
);
#6349=(
LENGTH_UNIT()
NAMED_UNIT(*)
SI_UNIT($,.METRE.)
);
#6350=(
NAMED_UNIT(*)
PLANE_ANGLE_UNIT()
SI_UNIT($,.RADIAN.)
);
#6351=(
NAMED_UNIT(*)
SI_UNIT($,.STERADIAN.)
SOLID_ANGLE_UNIT()
);
#6355=SHAPE_DEFINITION_REPRESENTATION(#6379,#6479);
#6379=PRODUCT_DEFINITION_SHAPE('',$,#6504);
#6479=SHAPE_REPRESENTATION('',(#3602),#6327);
#6500=PRODUCT_DEFINITION_CONTEXT('part definition',#6574,'design');
#6504=PRODUCT_DEFINITION('Front Left Z Mount','Front Left Z Mount',#6528,
#6500);
#6528=PRODUCT_DEFINITION_FORMATION('',$,#6579);
#6574=APPLICATION_CONTEXT('Managed model based 3d engineering');
#6575=PRODUCT_CONTEXT('part definition',#6574,'mechanical');
#6579=PRODUCT('Front Left Z Mount','Front Left Z Mount',
'LEGAL AND USAGE DISCLAIMER: this Data/Model is provided \X2\201C\X0\A
S IS\X2\201D\X0\ for informational and representational only. It is a 
geometric approximation and is NOT engineered, certified, or guarantee
d for dimensional accuracy, exact tolerances, or production-level prec
ision. Vendor disclaims all implied warranties including fitness for a
 particular purpose. DO NOT USE FOR DIRECT PHYSICAL MANUFACTURING, AUT
OMATED PRODUCTION, OR SAFETY-CRITICAL SYSTEMS without independent engi
neering verification and resolution of any design discrepancies.',(#6575));
#6602=PRESENTATION_STYLE_ASSIGNMENT((#6608));
#6608=SURFACE_STYLE_USAGE(.BOTH.,#6614);
#6614=SURFACE_SIDE_STYLE('',(#6620));
#6620=SURFACE_STYLE_FILL_AREA(#6626);
#6626=FILL_AREA_STYLE('Opaque(246,246,243)',(#6632));
#6632=FILL_AREA_STYLE_COLOUR('Opaque(246,246,243)',#6638);
#6638=COLOUR_RGB('Opaque(246,246,243)',0.964705882352941,0.964705882352941,
0.952941176470588);
ENDSEC;
END-ISO-10303-21;
